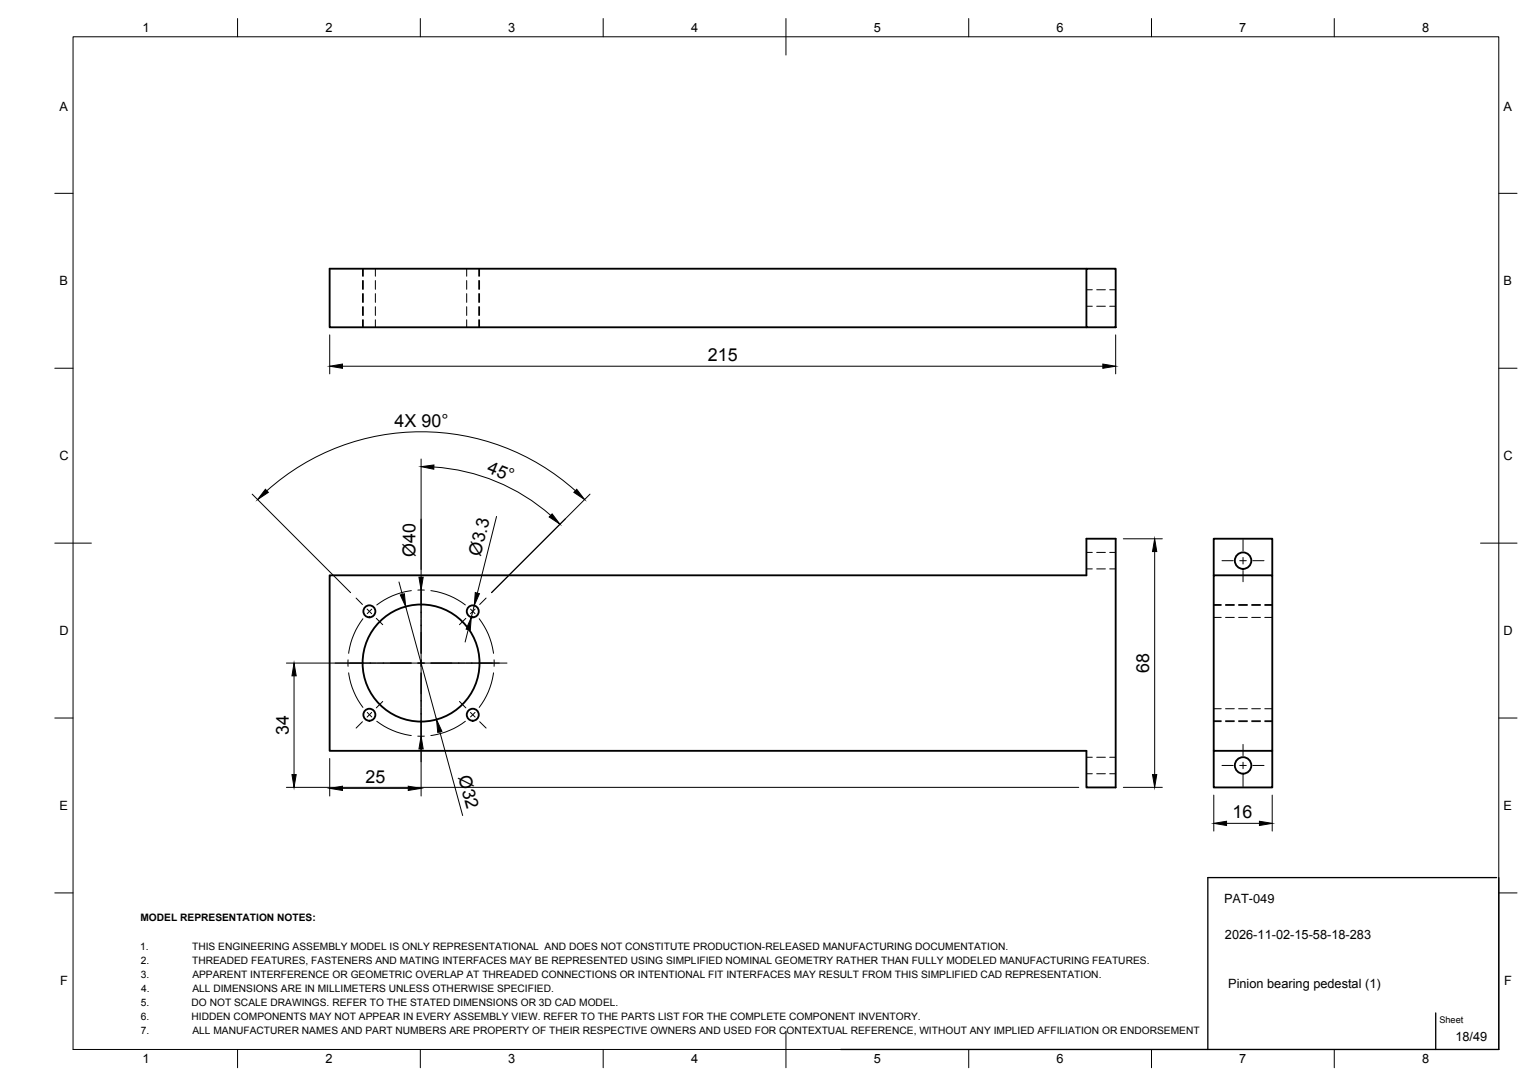
ISO-10303-21;
HEADER;
/* Generated by software containing ST-Developer
 * from STEP Tools, Inc. (www.steptools.com) 
 */

FILE_DESCRIPTION(
/* description */ ('Hand drill press frame (manual)'),
/* implementation_level */ '2;1');

FILE_NAME(
/* name */ 'Pinion bearing pedestal (1).step',
/* time_stamp */ '2026-10-28T03:25:28-07:00',
/* author */ (''),
/* organization */ (''),
/* preprocessor_version */ 'ST-DEVELOPER v20.2',
/* originating_system */ 'Autodesk Translation Framework v15.17.0.0',
/* authorisation */ '');

FILE_SCHEMA (('AUTOMOTIVE_DESIGN { 1 0 10303 214 3 1 1 }'));
ENDSEC;

DATA;
#10=MECHANICAL_DESIGN_GEOMETRIC_PRESENTATION_REPRESENTATION('',(#632),#33299);
#542=SHAPE_REPRESENTATION_RELATIONSHIP('SRR','None',#33501,#587);
#587=ADVANCED_BREP_SHAPE_REPRESENTATION('',(#684),#33263);
#632=STYLED_ITEM('',(#33814),#684);
#684=MANIFOLD_SOLID_BREP('Body1',#12650);
#800=FACE_BOUND('',#2292,.T.);
#801=FACE_BOUND('',#2294,.T.);
#802=FACE_BOUND('',#2298,.T.);
#803=FACE_BOUND('',#2299,.T.);
#804=FACE_BOUND('',#2300,.T.);
#805=FACE_BOUND('',#2301,.T.);
#806=FACE_BOUND('',#2302,.T.);
#807=FACE_BOUND('',#2305,.T.);
#808=FACE_BOUND('',#2306,.T.);
#809=FACE_BOUND('',#2307,.T.);
#810=FACE_BOUND('',#2308,.T.);
#811=FACE_BOUND('',#2309,.T.);
#812=FACE_BOUND('',#2313,.T.);
#813=FACE_BOUND('',#2314,.T.);
#999=PLANE('',#13535);
#1000=PLANE('',#13536);
#1001=PLANE('',#13537);
#1002=PLANE('',#13538);
#1003=PLANE('',#13539);
#1004=PLANE('',#13540);
#1005=PLANE('',#13541);
#1006=PLANE('',#13542);
#1007=PLANE('',#13543);
#1008=PLANE('',#13544);
#1515=FACE_OUTER_BOUND('',#2284,.T.);
#1516=FACE_OUTER_BOUND('',#2285,.T.);
#1517=FACE_OUTER_BOUND('',#2286,.T.);
#1518=FACE_OUTER_BOUND('',#2287,.T.);
#1519=FACE_OUTER_BOUND('',#2288,.T.);
#1520=FACE_OUTER_BOUND('',#2289,.T.);
#1521=FACE_OUTER_BOUND('',#2290,.T.);
#1522=FACE_OUTER_BOUND('',#2291,.T.);
#1523=FACE_OUTER_BOUND('',#2293,.T.);
#1524=FACE_OUTER_BOUND('',#2295,.T.);
#1525=FACE_OUTER_BOUND('',#2296,.T.);
#1526=FACE_OUTER_BOUND('',#2297,.T.);
#1527=FACE_OUTER_BOUND('',#2303,.T.);
#1528=FACE_OUTER_BOUND('',#2304,.T.);
#1529=FACE_OUTER_BOUND('',#2310,.T.);
#1530=FACE_OUTER_BOUND('',#2311,.T.);
#1531=FACE_OUTER_BOUND('',#2312,.T.);
#2284=EDGE_LOOP('',(#9263,#9264,#9265,#9266));
#2285=EDGE_LOOP('',(#9267,#9268,#9269,#9270));
#2286=EDGE_LOOP('',(#9271,#9272,#9273,#9274));
#2287=EDGE_LOOP('',(#9275,#9276,#9277,#9278));
#2288=EDGE_LOOP('',(#9279,#9280,#9281,#9282));
#2289=EDGE_LOOP('',(#9283,#9284,#9285,#9286));
#2290=EDGE_LOOP('',(#9287,#9288,#9289,#9290));
#2291=EDGE_LOOP('',(#9291,#9292,#9293,#9294));
#2292=EDGE_LOOP('',(#9295));
#2293=EDGE_LOOP('',(#9296,#9297,#9298,#9299));
#2294=EDGE_LOOP('',(#9300));
#2295=EDGE_LOOP('',(#9301,#9302,#9303,#9304));
#2296=EDGE_LOOP('',(#9305,#9306,#9307,#9308));
#2297=EDGE_LOOP('',(#9309,#9310,#9311,#9312,#9313,#9314,#9315,#9316));
#2298=EDGE_LOOP('',(#9317));
#2299=EDGE_LOOP('',(#9318));
#2300=EDGE_LOOP('',(#9319));
#2301=EDGE_LOOP('',(#9320));
#2302=EDGE_LOOP('',(#9321));
#2303=EDGE_LOOP('',(#9322,#9323,#9324,#9325));
#2304=EDGE_LOOP('',(#9326,#9327,#9328,#9329,#9330,#9331,#9332,#9333));
#2305=EDGE_LOOP('',(#9334));
#2306=EDGE_LOOP('',(#9335));
#2307=EDGE_LOOP('',(#9336));
#2308=EDGE_LOOP('',(#9337));
#2309=EDGE_LOOP('',(#9338));
#2310=EDGE_LOOP('',(#9339,#9340,#9341,#9342));
#2311=EDGE_LOOP('',(#9343,#9344,#9345,#9346));
#2312=EDGE_LOOP('',(#9347,#9348,#9349,#9350));
#2313=EDGE_LOOP('',(#9351));
#2314=EDGE_LOOP('',(#9352));
#3156=LINE('',#18971,#4321);
#3157=LINE('',#18977,#4322);
#3158=LINE('',#18983,#4323);
#3159=LINE('',#18989,#4324);
#3160=LINE('',#18995,#4325);
#3161=LINE('',#19001,#4326);
#3162=LINE('',#19007,#4327);
#3163=LINE('',#19012,#4328);
#3164=LINE('',#19014,#4329);
#3165=LINE('',#19016,#4330);
#3166=LINE('',#19017,#4331);
#3167=LINE('',#19021,#4332);
#3168=LINE('',#19023,#4333);
#3169=LINE('',#19025,#4334);
#3170=LINE('',#19026,#4335);
#3171=LINE('',#19029,#4336);
#3172=LINE('',#19031,#4337);
#3173=LINE('',#19032,#4338);
#3174=LINE('',#19035,#4339);
#3175=LINE('',#19037,#4340);
#3176=LINE('',#19038,#4341);
#3177=LINE('',#19041,#4342);
#3178=LINE('',#19043,#4343);
#3179=LINE('',#19044,#4344);
#3180=LINE('',#19045,#4345);
#3181=LINE('',#19048,#4346);
#3182=LINE('',#19049,#4347);
#3183=LINE('',#19052,#4348);
#3184=LINE('',#19053,#4349);
#3185=LINE('',#19054,#4350);
#3186=LINE('',#19056,#4351);
#4321=VECTOR('',#15295,0.165);
#4322=VECTOR('',#15302,0.165);
#4323=VECTOR('',#15309,0.165);
#4324=VECTOR('',#15316,0.165);
#4325=VECTOR('',#15323,0.225);
#4326=VECTOR('',#15330,0.225);
#4327=VECTOR('',#15337,1.6);
#4328=VECTOR('',#15342,1.);
#4329=VECTOR('',#15343,1.);
#4330=VECTOR('',#15344,1.);
#4331=VECTOR('',#15345,1.);
#4332=VECTOR('',#15348,1.);
#4333=VECTOR('',#15349,1.);
#4334=VECTOR('',#15350,1.);
#4335=VECTOR('',#15351,1.);
#4336=VECTOR('',#15354,1.);
#4337=VECTOR('',#15355,1.);
#4338=VECTOR('',#15356,1.);
#4339=VECTOR('',#15359,1.);
#4340=VECTOR('',#15360,1.);
#4341=VECTOR('',#15361,1.);
#4342=VECTOR('',#15364,1.);
#4343=VECTOR('',#15365,1.);
#4344=VECTOR('',#15366,1.);
#4345=VECTOR('',#15367,1.);
#4346=VECTOR('',#15370,1.);
#4347=VECTOR('',#15371,1.);
#4348=VECTOR('',#15374,1.);
#4349=VECTOR('',#15375,1.);
#4350=VECTOR('',#15376,1.);
#4351=VECTOR('',#15379,1.);
#5348=CIRCLE('',#13515,0.165);
#5349=CIRCLE('',#13516,0.165);
#5350=CIRCLE('',#13518,0.165);
#5351=CIRCLE('',#13519,0.165);
#5352=CIRCLE('',#13521,0.165);
#5353=CIRCLE('',#13522,0.165);
#5354=CIRCLE('',#13524,0.165);
#5355=CIRCLE('',#13525,0.165);
#5356=CIRCLE('',#13527,0.225);
#5357=CIRCLE('',#13528,0.225);
#5358=CIRCLE('',#13530,0.225);
#5359=CIRCLE('',#13531,0.225);
#5360=CIRCLE('',#13533,1.6);
#5361=CIRCLE('',#13534,1.6);
#5894=VERTEX_POINT('',#18968);
#5895=VERTEX_POINT('',#18970);
#5896=VERTEX_POINT('',#18974);
#5897=VERTEX_POINT('',#18976);
#5898=VERTEX_POINT('',#18980);
#5899=VERTEX_POINT('',#18982);
#5900=VERTEX_POINT('',#18986);
#5901=VERTEX_POINT('',#18988);
#5902=VERTEX_POINT('',#18992);
#5903=VERTEX_POINT('',#18994);
#5904=VERTEX_POINT('',#18998);
#5905=VERTEX_POINT('',#19000);
#5906=VERTEX_POINT('',#19004);
#5907=VERTEX_POINT('',#19006);
#5908=VERTEX_POINT('',#19010);
#5909=VERTEX_POINT('',#19011);
#5910=VERTEX_POINT('',#19013);
#5911=VERTEX_POINT('',#19015);
#5912=VERTEX_POINT('',#19019);
#5913=VERTEX_POINT('',#19020);
#5914=VERTEX_POINT('',#19022);
#5915=VERTEX_POINT('',#19024);
#5916=VERTEX_POINT('',#19028);
#5917=VERTEX_POINT('',#19030);
#5918=VERTEX_POINT('',#19034);
#5919=VERTEX_POINT('',#19036);
#5920=VERTEX_POINT('',#19040);
#5921=VERTEX_POINT('',#19042);
#5922=VERTEX_POINT('',#19047);
#5923=VERTEX_POINT('',#19051);
#7160=EDGE_CURVE('',#5894,#5894,#5348,.T.);
#7161=EDGE_CURVE('',#5894,#5895,#3156,.T.);
#7162=EDGE_CURVE('',#5895,#5895,#5349,.T.);
#7163=EDGE_CURVE('',#5896,#5896,#5350,.T.);
#7164=EDGE_CURVE('',#5896,#5897,#3157,.T.);
#7165=EDGE_CURVE('',#5897,#5897,#5351,.T.);
#7166=EDGE_CURVE('',#5898,#5898,#5352,.T.);
#7167=EDGE_CURVE('',#5898,#5899,#3158,.T.);
#7168=EDGE_CURVE('',#5899,#5899,#5353,.T.);
#7169=EDGE_CURVE('',#5900,#5900,#5354,.T.);
#7170=EDGE_CURVE('',#5900,#5901,#3159,.T.);
#7171=EDGE_CURVE('',#5901,#5901,#5355,.T.);
#7172=EDGE_CURVE('',#5902,#5902,#5356,.T.);
#7173=EDGE_CURVE('',#5902,#5903,#3160,.T.);
#7174=EDGE_CURVE('',#5903,#5903,#5357,.T.);
#7175=EDGE_CURVE('',#5904,#5904,#5358,.T.);
#7176=EDGE_CURVE('',#5904,#5905,#3161,.T.);
#7177=EDGE_CURVE('',#5905,#5905,#5359,.T.);
#7178=EDGE_CURVE('',#5906,#5906,#5360,.T.);
#7179=EDGE_CURVE('',#5906,#5907,#3162,.T.);
#7180=EDGE_CURVE('',#5907,#5907,#5361,.T.);
#7181=EDGE_CURVE('',#5908,#5909,#3163,.T.);
#7182=EDGE_CURVE('',#5910,#5908,#3164,.T.);
#7183=EDGE_CURVE('',#5910,#5911,#3165,.T.);
#7184=EDGE_CURVE('',#5909,#5911,#3166,.T.);
#7185=EDGE_CURVE('',#5912,#5913,#3167,.T.);
#7186=EDGE_CURVE('',#5914,#5912,#3168,.T.);
#7187=EDGE_CURVE('',#5915,#5914,#3169,.T.);
#7188=EDGE_CURVE('',#5913,#5915,#3170,.T.);
#7189=EDGE_CURVE('',#5915,#5916,#3171,.T.);
#7190=EDGE_CURVE('',#5917,#5914,#3172,.T.);
#7191=EDGE_CURVE('',#5916,#5917,#3173,.T.);
#7192=EDGE_CURVE('',#5918,#5910,#3174,.T.);
#7193=EDGE_CURVE('',#5918,#5919,#3175,.T.);
#7194=EDGE_CURVE('',#5911,#5919,#3176,.T.);
#7195=EDGE_CURVE('',#5908,#5920,#3177,.T.);
#7196=EDGE_CURVE('',#5921,#5920,#3178,.T.);
#7197=EDGE_CURVE('',#5913,#5921,#3179,.T.);
#7198=EDGE_CURVE('',#5916,#5918,#3180,.T.);
#7199=EDGE_CURVE('',#5909,#5922,#3181,.T.);
#7200=EDGE_CURVE('',#5920,#5922,#3182,.T.);
#7201=EDGE_CURVE('',#5912,#5923,#3183,.T.);
#7202=EDGE_CURVE('',#5922,#5923,#3184,.T.);
#7203=EDGE_CURVE('',#5919,#5917,#3185,.T.);
#7204=EDGE_CURVE('',#5923,#5921,#3186,.T.);
#9263=ORIENTED_EDGE('',*,*,#7160,.F.);
#9264=ORIENTED_EDGE('',*,*,#7161,.T.);
#9265=ORIENTED_EDGE('',*,*,#7162,.F.);
#9266=ORIENTED_EDGE('',*,*,#7161,.F.);
#9267=ORIENTED_EDGE('',*,*,#7163,.F.);
#9268=ORIENTED_EDGE('',*,*,#7164,.T.);
#9269=ORIENTED_EDGE('',*,*,#7165,.F.);
#9270=ORIENTED_EDGE('',*,*,#7164,.F.);
#9271=ORIENTED_EDGE('',*,*,#7166,.F.);
#9272=ORIENTED_EDGE('',*,*,#7167,.T.);
#9273=ORIENTED_EDGE('',*,*,#7168,.F.);
#9274=ORIENTED_EDGE('',*,*,#7167,.F.);
#9275=ORIENTED_EDGE('',*,*,#7169,.F.);
#9276=ORIENTED_EDGE('',*,*,#7170,.T.);
#9277=ORIENTED_EDGE('',*,*,#7171,.F.);
#9278=ORIENTED_EDGE('',*,*,#7170,.F.);
#9279=ORIENTED_EDGE('',*,*,#7172,.F.);
#9280=ORIENTED_EDGE('',*,*,#7173,.T.);
#9281=ORIENTED_EDGE('',*,*,#7174,.F.);
#9282=ORIENTED_EDGE('',*,*,#7173,.F.);
#9283=ORIENTED_EDGE('',*,*,#7175,.F.);
#9284=ORIENTED_EDGE('',*,*,#7176,.T.);
#9285=ORIENTED_EDGE('',*,*,#7177,.F.);
#9286=ORIENTED_EDGE('',*,*,#7176,.F.);
#9287=ORIENTED_EDGE('',*,*,#7178,.F.);
#9288=ORIENTED_EDGE('',*,*,#7179,.T.);
#9289=ORIENTED_EDGE('',*,*,#7180,.F.);
#9290=ORIENTED_EDGE('',*,*,#7179,.F.);
#9291=ORIENTED_EDGE('',*,*,#7181,.F.);
#9292=ORIENTED_EDGE('',*,*,#7182,.F.);
#9293=ORIENTED_EDGE('',*,*,#7183,.T.);
#9294=ORIENTED_EDGE('',*,*,#7184,.F.);
#9295=ORIENTED_EDGE('',*,*,#7177,.T.);
#9296=ORIENTED_EDGE('',*,*,#7185,.F.);
#9297=ORIENTED_EDGE('',*,*,#7186,.F.);
#9298=ORIENTED_EDGE('',*,*,#7187,.F.);
#9299=ORIENTED_EDGE('',*,*,#7188,.F.);
#9300=ORIENTED_EDGE('',*,*,#7174,.T.);
#9301=ORIENTED_EDGE('',*,*,#7189,.F.);
#9302=ORIENTED_EDGE('',*,*,#7187,.T.);
#9303=ORIENTED_EDGE('',*,*,#7190,.F.);
#9304=ORIENTED_EDGE('',*,*,#7191,.F.);
#9305=ORIENTED_EDGE('',*,*,#7192,.F.);
#9306=ORIENTED_EDGE('',*,*,#7193,.T.);
#9307=ORIENTED_EDGE('',*,*,#7194,.F.);
#9308=ORIENTED_EDGE('',*,*,#7183,.F.);
#9309=ORIENTED_EDGE('',*,*,#7195,.T.);
#9310=ORIENTED_EDGE('',*,*,#7196,.F.);
#9311=ORIENTED_EDGE('',*,*,#7197,.F.);
#9312=ORIENTED_EDGE('',*,*,#7188,.T.);
#9313=ORIENTED_EDGE('',*,*,#7189,.T.);
#9314=ORIENTED_EDGE('',*,*,#7198,.T.);
#9315=ORIENTED_EDGE('',*,*,#7192,.T.);
#9316=ORIENTED_EDGE('',*,*,#7182,.T.);
#9317=ORIENTED_EDGE('',*,*,#7178,.T.);
#9318=ORIENTED_EDGE('',*,*,#7169,.T.);
#9319=ORIENTED_EDGE('',*,*,#7166,.T.);
#9320=ORIENTED_EDGE('',*,*,#7163,.T.);
#9321=ORIENTED_EDGE('',*,*,#7160,.T.);
#9322=ORIENTED_EDGE('',*,*,#7181,.T.);
#9323=ORIENTED_EDGE('',*,*,#7199,.T.);
#9324=ORIENTED_EDGE('',*,*,#7200,.F.);
#9325=ORIENTED_EDGE('',*,*,#7195,.F.);
#9326=ORIENTED_EDGE('',*,*,#7201,.T.);
#9327=ORIENTED_EDGE('',*,*,#7202,.F.);
#9328=ORIENTED_EDGE('',*,*,#7199,.F.);
#9329=ORIENTED_EDGE('',*,*,#7184,.T.);
#9330=ORIENTED_EDGE('',*,*,#7194,.T.);
#9331=ORIENTED_EDGE('',*,*,#7203,.T.);
#9332=ORIENTED_EDGE('',*,*,#7190,.T.);
#9333=ORIENTED_EDGE('',*,*,#7186,.T.);
#9334=ORIENTED_EDGE('',*,*,#7180,.T.);
#9335=ORIENTED_EDGE('',*,*,#7171,.T.);
#9336=ORIENTED_EDGE('',*,*,#7168,.T.);
#9337=ORIENTED_EDGE('',*,*,#7165,.T.);
#9338=ORIENTED_EDGE('',*,*,#7162,.T.);
#9339=ORIENTED_EDGE('',*,*,#7185,.T.);
#9340=ORIENTED_EDGE('',*,*,#7197,.T.);
#9341=ORIENTED_EDGE('',*,*,#7204,.F.);
#9342=ORIENTED_EDGE('',*,*,#7201,.F.);
#9343=ORIENTED_EDGE('',*,*,#7204,.T.);
#9344=ORIENTED_EDGE('',*,*,#7196,.T.);
#9345=ORIENTED_EDGE('',*,*,#7200,.T.);
#9346=ORIENTED_EDGE('',*,*,#7202,.T.);
#9347=ORIENTED_EDGE('',*,*,#7203,.F.);
#9348=ORIENTED_EDGE('',*,*,#7193,.F.);
#9349=ORIENTED_EDGE('',*,*,#7198,.F.);
#9350=ORIENTED_EDGE('',*,*,#7191,.T.);
#9351=ORIENTED_EDGE('',*,*,#7172,.T.);
#9352=ORIENTED_EDGE('',*,*,#7175,.T.);
#11849=CYLINDRICAL_SURFACE('',#13514,0.165);
#11850=CYLINDRICAL_SURFACE('',#13517,0.165);
#11851=CYLINDRICAL_SURFACE('',#13520,0.165);
#11852=CYLINDRICAL_SURFACE('',#13523,0.165);
#11853=CYLINDRICAL_SURFACE('',#13526,0.225);
#11854=CYLINDRICAL_SURFACE('',#13529,0.225);
#11855=CYLINDRICAL_SURFACE('',#13532,1.6);
#12124=ADVANCED_FACE('',(#1515),#11849,.F.);
#12125=ADVANCED_FACE('',(#1516),#11850,.F.);
#12126=ADVANCED_FACE('',(#1517),#11851,.F.);
#12127=ADVANCED_FACE('',(#1518),#11852,.F.);
#12128=ADVANCED_FACE('',(#1519),#11853,.F.);
#12129=ADVANCED_FACE('',(#1520),#11854,.F.);
#12130=ADVANCED_FACE('',(#1521),#11855,.F.);
#12131=ADVANCED_FACE('',(#1522,#800),#999,.T.);
#12132=ADVANCED_FACE('',(#1523,#801),#1000,.T.);
#12133=ADVANCED_FACE('',(#1524),#1001,.T.);
#12134=ADVANCED_FACE('',(#1525),#1002,.T.);
#12135=ADVANCED_FACE('',(#1526,#802,#803,#804,#805,#806),#1003,.T.);
#12136=ADVANCED_FACE('',(#1527),#1004,.T.);
#12137=ADVANCED_FACE('',(#1528,#807,#808,#809,#810,#811),#1005,.T.);
#12138=ADVANCED_FACE('',(#1529),#1006,.T.);
#12139=ADVANCED_FACE('',(#1530),#1007,.T.);
#12140=ADVANCED_FACE('',(#1531,#812,#813),#1008,.F.);
#12650=CLOSED_SHELL('',(#12124,#12125,#12126,#12127,#12128,#12129,#12130,
#12131,#12132,#12133,#12134,#12135,#12136,#12137,#12138,#12139,#12140));
#13513=AXIS2_PLACEMENT_3D('',#18966,#15289,#15290);
#13514=AXIS2_PLACEMENT_3D('',#18967,#15291,#15292);
#13515=AXIS2_PLACEMENT_3D('',#18969,#15293,#15294);
#13516=AXIS2_PLACEMENT_3D('',#18972,#15296,#15297);
#13517=AXIS2_PLACEMENT_3D('',#18973,#15298,#15299);
#13518=AXIS2_PLACEMENT_3D('',#18975,#15300,#15301);
#13519=AXIS2_PLACEMENT_3D('',#18978,#15303,#15304);
#13520=AXIS2_PLACEMENT_3D('',#18979,#15305,#15306);
#13521=AXIS2_PLACEMENT_3D('',#18981,#15307,#15308);
#13522=AXIS2_PLACEMENT_3D('',#18984,#15310,#15311);
#13523=AXIS2_PLACEMENT_3D('',#18985,#15312,#15313);
#13524=AXIS2_PLACEMENT_3D('',#18987,#15314,#15315);
#13525=AXIS2_PLACEMENT_3D('',#18990,#15317,#15318);
#13526=AXIS2_PLACEMENT_3D('',#18991,#15319,#15320);
#13527=AXIS2_PLACEMENT_3D('',#18993,#15321,#15322);
#13528=AXIS2_PLACEMENT_3D('',#18996,#15324,#15325);
#13529=AXIS2_PLACEMENT_3D('',#18997,#15326,#15327);
#13530=AXIS2_PLACEMENT_3D('',#18999,#15328,#15329);
#13531=AXIS2_PLACEMENT_3D('',#19002,#15331,#15332);
#13532=AXIS2_PLACEMENT_3D('',#19003,#15333,#15334);
#13533=AXIS2_PLACEMENT_3D('',#19005,#15335,#15336);
#13534=AXIS2_PLACEMENT_3D('',#19008,#15338,#15339);
#13535=AXIS2_PLACEMENT_3D('',#19009,#15340,#15341);
#13536=AXIS2_PLACEMENT_3D('',#19018,#15346,#15347);
#13537=AXIS2_PLACEMENT_3D('',#19027,#15352,#15353);
#13538=AXIS2_PLACEMENT_3D('',#19033,#15357,#15358);
#13539=AXIS2_PLACEMENT_3D('',#19039,#15362,#15363);
#13540=AXIS2_PLACEMENT_3D('',#19046,#15368,#15369);
#13541=AXIS2_PLACEMENT_3D('',#19050,#15372,#15373);
#13542=AXIS2_PLACEMENT_3D('',#19055,#15377,#15378);
#13543=AXIS2_PLACEMENT_3D('',#19057,#15380,#15381);
#13544=AXIS2_PLACEMENT_3D('',#19058,#15382,#15383);
#15289=DIRECTION('axis',(0.,0.,1.));
#15290=DIRECTION('refdir',(1.,0.,0.));
#15291=DIRECTION('center_axis',(0.,1.,0.));
#15292=DIRECTION('ref_axis',(1.,0.,0.));
#15293=DIRECTION('center_axis',(0.,1.,0.));
#15294=DIRECTION('ref_axis',(1.,0.,0.));
#15295=DIRECTION('',(0.,1.,0.));
#15296=DIRECTION('center_axis',(0.,-1.,0.));
#15297=DIRECTION('ref_axis',(1.,0.,0.));
#15298=DIRECTION('center_axis',(0.,1.,0.));
#15299=DIRECTION('ref_axis',(1.,0.,0.));
#15300=DIRECTION('center_axis',(0.,1.,0.));
#15301=DIRECTION('ref_axis',(1.,0.,0.));
#15302=DIRECTION('',(0.,1.,0.));
#15303=DIRECTION('center_axis',(0.,-1.,0.));
#15304=DIRECTION('ref_axis',(1.,0.,0.));
#15305=DIRECTION('center_axis',(0.,1.,0.));
#15306=DIRECTION('ref_axis',(1.,0.,0.));
#15307=DIRECTION('center_axis',(0.,1.,0.));
#15308=DIRECTION('ref_axis',(1.,0.,0.));
#15309=DIRECTION('',(0.,1.,0.));
#15310=DIRECTION('center_axis',(0.,-1.,0.));
#15311=DIRECTION('ref_axis',(1.,0.,0.));
#15312=DIRECTION('center_axis',(0.,1.,0.));
#15313=DIRECTION('ref_axis',(1.,0.,0.));
#15314=DIRECTION('center_axis',(0.,1.,0.));
#15315=DIRECTION('ref_axis',(1.,0.,0.));
#15316=DIRECTION('',(0.,1.,0.));
#15317=DIRECTION('center_axis',(0.,-1.,0.));
#15318=DIRECTION('ref_axis',(1.,0.,0.));
#15319=DIRECTION('center_axis',(0.,0.,1.));
#15320=DIRECTION('ref_axis',(1.,0.,0.));
#15321=DIRECTION('center_axis',(0.,0.,1.));
#15322=DIRECTION('ref_axis',(1.,0.,0.));
#15323=DIRECTION('',(0.,0.,1.));
#15324=DIRECTION('center_axis',(0.,0.,-1.));
#15325=DIRECTION('ref_axis',(1.,0.,0.));
#15326=DIRECTION('center_axis',(0.,0.,1.));
#15327=DIRECTION('ref_axis',(1.,0.,0.));
#15328=DIRECTION('center_axis',(0.,0.,1.));
#15329=DIRECTION('ref_axis',(1.,0.,0.));
#15330=DIRECTION('',(0.,0.,1.));
#15331=DIRECTION('center_axis',(0.,0.,-1.));
#15332=DIRECTION('ref_axis',(1.,0.,0.));
#15333=DIRECTION('center_axis',(0.,1.,0.));
#15334=DIRECTION('ref_axis',(1.,0.,0.));
#15335=DIRECTION('center_axis',(0.,1.,0.));
#15336=DIRECTION('ref_axis',(1.,0.,0.));
#15337=DIRECTION('',(0.,1.,0.));
#15338=DIRECTION('center_axis',(0.,-1.,0.));
#15339=DIRECTION('ref_axis',(1.,0.,0.));
#15340=DIRECTION('center_axis',(0.,0.,1.));
#15341=DIRECTION('ref_axis',(1.,0.,0.));
#15342=DIRECTION('',(0.,1.,0.));
#15343=DIRECTION('',(-1.,0.,0.));
#15344=DIRECTION('',(0.,1.,0.));
#15345=DIRECTION('',(1.,0.,0.));
#15346=DIRECTION('center_axis',(0.,0.,1.));
#15347=DIRECTION('ref_axis',(1.,0.,0.));
#15348=DIRECTION('',(0.,-1.,0.));
#15349=DIRECTION('',(1.,0.,0.));
#15350=DIRECTION('',(0.,1.,0.));
#15351=DIRECTION('',(-1.,0.,0.));
#15352=DIRECTION('center_axis',(-1.,0.,0.));
#15353=DIRECTION('ref_axis',(0.,0.,1.));
#15354=DIRECTION('',(0.,0.,-1.));
#15355=DIRECTION('',(0.,0.,1.));
#15356=DIRECTION('',(0.,1.,0.));
#15357=DIRECTION('center_axis',(1.,0.,0.));
#15358=DIRECTION('ref_axis',(0.,0.,-1.));
#15359=DIRECTION('',(0.,0.,1.));
#15360=DIRECTION('',(0.,1.,0.));
#15361=DIRECTION('',(0.,0.,-1.));
#15362=DIRECTION('center_axis',(0.,-1.,0.));
#15363=DIRECTION('ref_axis',(1.,0.,0.));
#15364=DIRECTION('',(0.,0.,1.));
#15365=DIRECTION('',(1.,0.,0.));
#15366=DIRECTION('',(0.,0.,1.));
#15367=DIRECTION('',(1.,0.,0.));
#15368=DIRECTION('center_axis',(1.,0.,0.));
#15369=DIRECTION('ref_axis',(0.,1.,0.));
#15370=DIRECTION('',(0.,0.,1.));
#15371=DIRECTION('',(0.,1.,0.));
#15372=DIRECTION('center_axis',(0.,1.,0.));
#15373=DIRECTION('ref_axis',(-1.,0.,0.));
#15374=DIRECTION('',(0.,0.,1.));
#15375=DIRECTION('',(-1.,0.,0.));
#15376=DIRECTION('',(-1.,0.,0.));
#15377=DIRECTION('center_axis',(-1.,0.,0.));
#15378=DIRECTION('ref_axis',(0.,-1.,0.));
#15379=DIRECTION('',(0.,-1.,0.));
#15380=DIRECTION('center_axis',(0.,0.,1.));
#15381=DIRECTION('ref_axis',(1.,0.,0.));
#15382=DIRECTION('center_axis',(0.,0.,1.));
#15383=DIRECTION('ref_axis',(1.,0.,0.));
#18966=CARTESIAN_POINT('',(0.,0.,0.));
#18967=CARTESIAN_POINT('Origin',(-4.66421356237309,2.1,18.5857864376269));
#18968=CARTESIAN_POINT('',(-4.82921356237309,2.2,18.5857864376269));
#18969=CARTESIAN_POINT('Origin',(-4.66421356237309,2.2,18.5857864376269));
#18970=CARTESIAN_POINT('',(-4.82921356237309,3.8,18.5857864376269));
#18971=CARTESIAN_POINT('',(-4.82921356237309,2.1,18.5857864376269));
#18972=CARTESIAN_POINT('Origin',(-4.66421356237309,3.8,18.5857864376269));
#18973=CARTESIAN_POINT('Origin',(-4.66421356237309,2.1,21.4142135623731));
#18974=CARTESIAN_POINT('',(-4.82921356237309,2.2,21.4142135623731));
#18975=CARTESIAN_POINT('Origin',(-4.66421356237309,2.2,21.4142135623731));
#18976=CARTESIAN_POINT('',(-4.82921356237309,3.8,21.4142135623731));
#18977=CARTESIAN_POINT('',(-4.82921356237309,2.1,21.4142135623731));
#18978=CARTESIAN_POINT('Origin',(-4.66421356237309,3.8,21.4142135623731));
#18979=CARTESIAN_POINT('Origin',(-1.8357864376269,2.1,21.4142135623731));
#18980=CARTESIAN_POINT('',(-2.00078643762691,2.2,21.4142135623731));
#18981=CARTESIAN_POINT('Origin',(-1.8357864376269,2.2,21.4142135623731));
#18982=CARTESIAN_POINT('',(-2.00078643762691,3.8,21.4142135623731));
#18983=CARTESIAN_POINT('',(-2.00078643762691,2.1,21.4142135623731));
#18984=CARTESIAN_POINT('Origin',(-1.8357864376269,3.8,21.4142135623731));
#18985=CARTESIAN_POINT('Origin',(-1.83578643762691,2.1,18.5857864376269));
#18986=CARTESIAN_POINT('',(-2.00078643762691,2.2,18.5857864376269));
#18987=CARTESIAN_POINT('Origin',(-1.83578643762691,2.2,18.5857864376269));
#18988=CARTESIAN_POINT('',(-2.00078643762691,3.8,18.5857864376269));
#18989=CARTESIAN_POINT('',(-2.00078643762691,2.1,18.5857864376269));
#18990=CARTESIAN_POINT('Origin',(-1.83578643762691,3.8,18.5857864376269));
#18991=CARTESIAN_POINT('Origin',(-6.05,3.,0.9));
#18992=CARTESIAN_POINT('',(-6.275,3.,1.));
#18993=CARTESIAN_POINT('Origin',(-6.05,3.,1.));
#18994=CARTESIAN_POINT('',(-6.275,3.,1.8));
#18995=CARTESIAN_POINT('',(-6.275,3.,0.9));
#18996=CARTESIAN_POINT('Origin',(-6.05,3.,1.8));
#18997=CARTESIAN_POINT('Origin',(-0.45,3.,0.9));
#18998=CARTESIAN_POINT('',(-0.675,3.,1.));
#18999=CARTESIAN_POINT('Origin',(-0.45,3.,1.));
#19000=CARTESIAN_POINT('',(-0.675,3.,1.8));
#19001=CARTESIAN_POINT('',(-0.675,3.,0.9));
#19002=CARTESIAN_POINT('Origin',(-0.45,3.,1.8));
#19003=CARTESIAN_POINT('Origin',(-3.25,2.1,20.));
#19004=CARTESIAN_POINT('',(-4.85,2.2,20.));
#19005=CARTESIAN_POINT('Origin',(-3.25,2.2,20.));
#19006=CARTESIAN_POINT('',(-4.85,3.8,20.));
#19007=CARTESIAN_POINT('',(-4.85,2.1,20.));
#19008=CARTESIAN_POINT('Origin',(-3.25,3.8,20.));
#19009=CARTESIAN_POINT('Origin',(-6.65,2.2,1.8));
#19010=CARTESIAN_POINT('',(-0.85,2.2,1.8));
#19011=CARTESIAN_POINT('',(-0.85,3.8,1.8));
#19012=CARTESIAN_POINT('',(-0.85,2.2,1.8));
#19013=CARTESIAN_POINT('',(0.15,2.2,1.8));
#19014=CARTESIAN_POINT('',(0.15,2.2,1.8));
#19015=CARTESIAN_POINT('',(0.15,3.8,1.8));
#19016=CARTESIAN_POINT('',(0.15,2.2,1.8));
#19017=CARTESIAN_POINT('',(0.15,3.8,1.8));
#19018=CARTESIAN_POINT('Origin',(-6.65,2.2,1.8));
#19019=CARTESIAN_POINT('',(-5.65,3.8,1.8));
#19020=CARTESIAN_POINT('',(-5.65,2.2,1.8));
#19021=CARTESIAN_POINT('',(-5.65,3.,1.8));
#19022=CARTESIAN_POINT('',(-6.65,3.8,1.8));
#19023=CARTESIAN_POINT('',(0.15,3.8,1.8));
#19024=CARTESIAN_POINT('',(-6.65,2.2,1.8));
#19025=CARTESIAN_POINT('',(-6.65,2.2,1.8));
#19026=CARTESIAN_POINT('',(0.15,2.2,1.8));
#19027=CARTESIAN_POINT('Origin',(-6.65,2.2,1.));
#19028=CARTESIAN_POINT('',(-6.65,2.2,1.));
#19029=CARTESIAN_POINT('',(-6.65,2.2,1.8));
#19030=CARTESIAN_POINT('',(-6.65,3.8,1.));
#19031=CARTESIAN_POINT('',(-6.65,3.8,1.8));
#19032=CARTESIAN_POINT('',(-6.65,2.2,1.));
#19033=CARTESIAN_POINT('Origin',(0.15,2.2,1.8));
#19034=CARTESIAN_POINT('',(0.15,2.2,1.));
#19035=CARTESIAN_POINT('',(0.15,2.2,1.));
#19036=CARTESIAN_POINT('',(0.15,3.8,1.));
#19037=CARTESIAN_POINT('',(0.15,2.2,1.));
#19038=CARTESIAN_POINT('',(0.15,3.8,1.));
#19039=CARTESIAN_POINT('Origin',(-5.65,2.2,1.));
#19040=CARTESIAN_POINT('',(-0.85,2.2,22.5));
#19041=CARTESIAN_POINT('',(-0.85,2.2,1.));
#19042=CARTESIAN_POINT('',(-5.65,2.2,22.5));
#19043=CARTESIAN_POINT('',(-5.65,2.2,22.5));
#19044=CARTESIAN_POINT('',(-5.65,2.2,1.));
#19045=CARTESIAN_POINT('',(-6.65,2.2,1.));
#19046=CARTESIAN_POINT('Origin',(-0.85,2.2,1.));
#19047=CARTESIAN_POINT('',(-0.85,3.8,22.5));
#19048=CARTESIAN_POINT('',(-0.85,3.8,1.));
#19049=CARTESIAN_POINT('',(-0.85,2.2,22.5));
#19050=CARTESIAN_POINT('Origin',(-0.85,3.8,1.));
#19051=CARTESIAN_POINT('',(-5.65,3.8,22.5));
#19052=CARTESIAN_POINT('',(-5.65,3.8,1.));
#19053=CARTESIAN_POINT('',(-0.85,3.8,22.5));
#19054=CARTESIAN_POINT('',(-6.65,3.8,1.));
#19055=CARTESIAN_POINT('Origin',(-5.65,3.8,1.));
#19056=CARTESIAN_POINT('',(-5.65,3.8,22.5));
#19057=CARTESIAN_POINT('Origin',(-3.25,3.,22.5));
#19058=CARTESIAN_POINT('Origin',(-3.25,3.,1.));
#33211=UNCERTAINTY_MEASURE_WITH_UNIT(LENGTH_MEASURE(0.001),#33300,
'DISTANCE_ACCURACY_VALUE',
'Maximum model space distance between geometric entities at asserted c
onnectivities');
#33247=UNCERTAINTY_MEASURE_WITH_UNIT(LENGTH_MEASURE(0.001),#33300,
'DISTANCE_ACCURACY_VALUE',
'Maximum model space distance between geometric entities at asserted c
onnectivities');
#33263=(
GEOMETRIC_REPRESENTATION_CONTEXT(3)
GLOBAL_UNCERTAINTY_ASSIGNED_CONTEXT((#33211))
GLOBAL_UNIT_ASSIGNED_CONTEXT((#33300,#33302,#33303))
REPRESENTATION_CONTEXT('','3D')
);
#33299=(
GEOMETRIC_REPRESENTATION_CONTEXT(3)
GLOBAL_UNCERTAINTY_ASSIGNED_CONTEXT((#33247))
GLOBAL_UNIT_ASSIGNED_CONTEXT((#33300,#33302,#33303))
REPRESENTATION_CONTEXT('','3D')
);
#33300=(
LENGTH_UNIT()
NAMED_UNIT(*)
SI_UNIT(.CENTI.,.METRE.)
);
#33302=(
NAMED_UNIT(*)
PLANE_ANGLE_UNIT()
SI_UNIT($,.RADIAN.)
);
#33303=(
NAMED_UNIT(*)
SI_UNIT($,.STERADIAN.)
SOLID_ANGLE_UNIT()
);
#33319=SHAPE_DEFINITION_REPRESENTATION(#33370,#33501);
#33370=PRODUCT_DEFINITION_SHAPE('',$,#33553);
#33501=SHAPE_REPRESENTATION('',(#13513),#33263);
#33537=PRODUCT_DEFINITION_CONTEXT('part definition',#33692,'design');
#33553=PRODUCT_DEFINITION('Pinion bearing pedestal (1)',
'Pinion bearing pedestal (1)',#33604,#33537);
#33604=PRODUCT_DEFINITION_FORMATION('',$,#33709);
#33692=APPLICATION_CONTEXT(
'Core Data for Automotive Mechanical Design Process');
#33693=PRODUCT_CONTEXT('part definition',#33692,'mechanical');
#33709=PRODUCT('Pinion bearing pedestal (1)',
'Pinion bearing pedestal (1)','Pinion bearing pedestal (1)',(#33693));
#33808=COLOUR_RGB('Grey',0.48,0.52,0.57);
#33809=FILL_AREA_STYLE_COLOUR('',#33808);
#33810=FILL_AREA_STYLE('',(#33809));
#33811=SURFACE_STYLE_FILL_AREA(#33810);
#33812=SURFACE_SIDE_STYLE('',(#33811));
#33813=SURFACE_STYLE_USAGE(.BOTH.,#33812);
#33814=PRESENTATION_STYLE_ASSIGNMENT((#33813));
ENDSEC;
END-ISO-10303-21;
